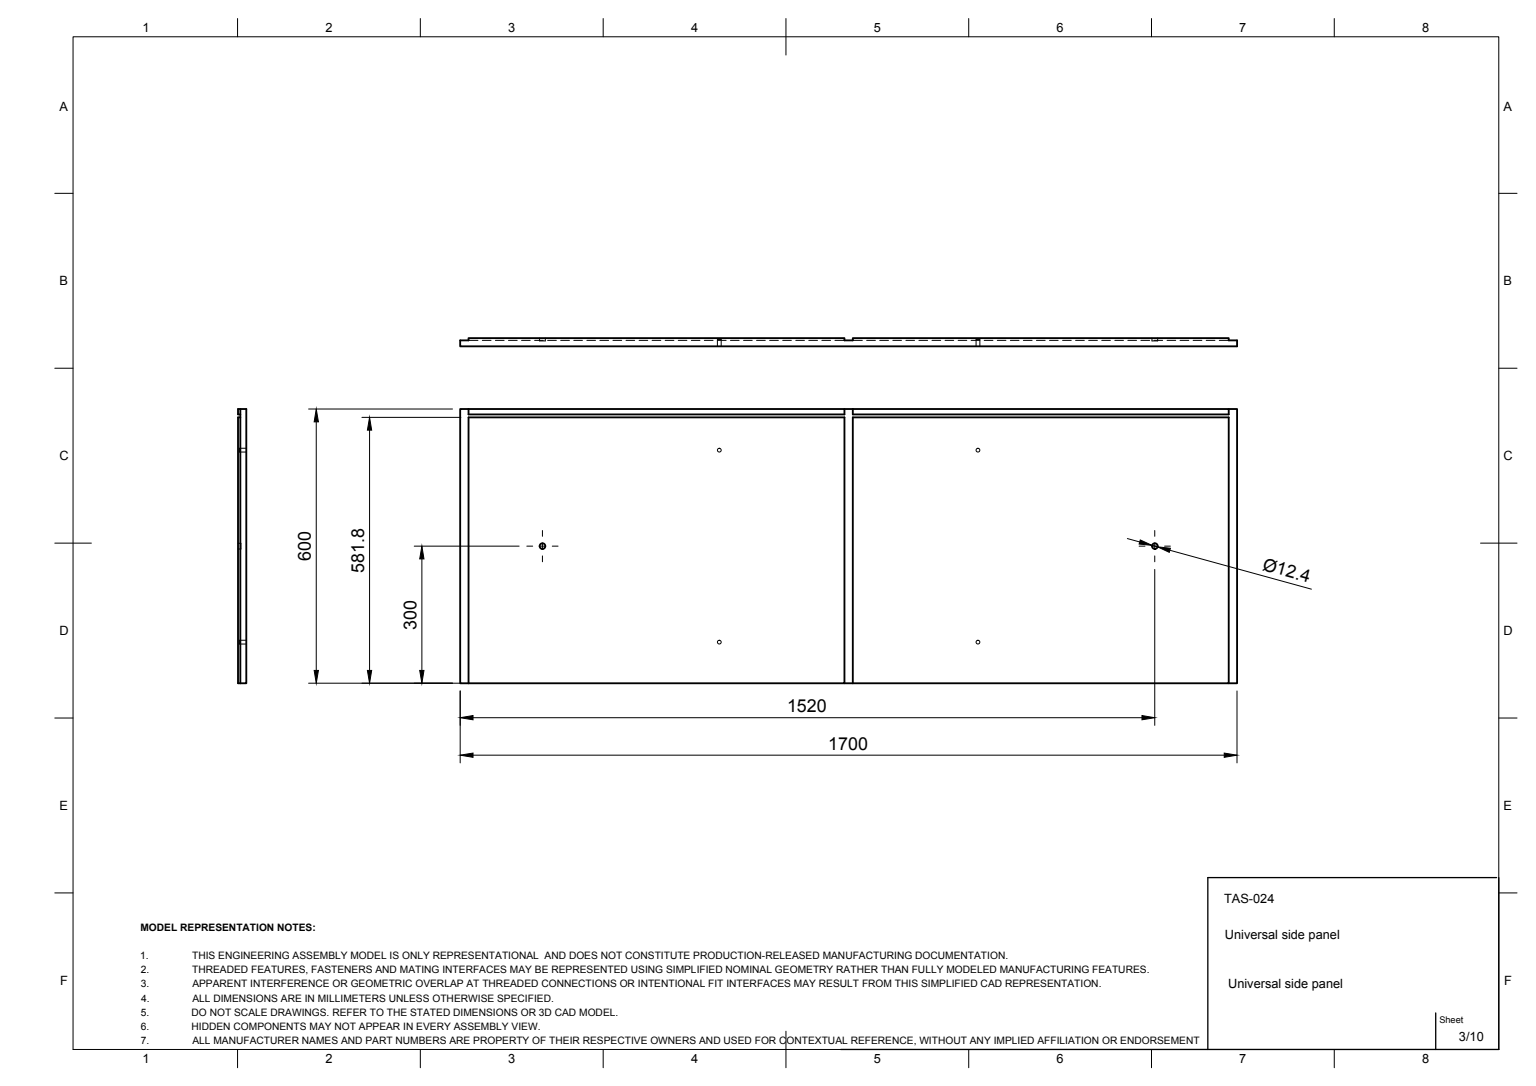
ISO-10303-21;
HEADER;
/* Generated by software containing ST-Developer
 * from STEP Tools, Inc. (www.steptools.com) 
 */

FILE_DESCRIPTION(
/* description */ (''),
/* implementation_level */ '2;1');

FILE_NAME(
/* name */ 'Universal side panel.step',
/* time_stamp */ '2026-11-15T17:53:25-08:00',
/* author */ (''),
/* organization */ (''),
/* preprocessor_version */ 'ST-DEVELOPER v20.2',
/* originating_system */ 'Autodesk Translation Framework v15.17.0.0',
/* authorisation */ '');

FILE_SCHEMA (('AUTOMOTIVE_DESIGN { 1 0 10303 214 3 1 1 }'));
ENDSEC;

DATA;
#10=MECHANICAL_DESIGN_GEOMETRIC_PRESENTATION_REPRESENTATION('',(#131),#2673);
#115=SHAPE_REPRESENTATION_RELATIONSHIP('SRR','None',#2723,#123);
#123=ADVANCED_BREP_SHAPE_REPRESENTATION('',(#139),#2665);
#131=STYLED_ITEM('',(#2772),#139);
#139=MANIFOLD_SOLID_BREP('Body1',#1517);
#147=FACE_BOUND('',#342,.T.);
#148=FACE_BOUND('',#349,.T.);
#149=FACE_BOUND('',#357,.T.);
#150=FACE_BOUND('',#358,.T.);
#151=FACE_BOUND('',#359,.T.);
#152=FACE_BOUND('',#360,.T.);
#160=PLANE('',#1619);
#161=PLANE('',#1623);
#162=PLANE('',#1627);
#163=PLANE('',#1631);
#164=PLANE('',#1635);
#165=PLANE('',#1639);
#166=PLANE('',#1640);
#167=PLANE('',#1641);
#168=PLANE('',#1642);
#169=PLANE('',#1643);
#170=PLANE('',#1644);
#171=PLANE('',#1645);
#172=PLANE('',#1646);
#173=PLANE('',#1647);
#174=PLANE('',#1648);
#175=PLANE('',#1649);
#176=PLANE('',#1650);
#177=PLANE('',#1651);
#178=PLANE('',#1652);
#179=PLANE('',#1653);
#180=PLANE('',#1654);
#181=PLANE('',#1655);
#182=PLANE('',#1656);
#183=PLANE('',#1657);
#184=PLANE('',#1658);
#185=PLANE('',#1659);
#186=PLANE('',#1660);
#187=PLANE('',#1661);
#233=FACE_OUTER_BOUND('',#322,.T.);
#234=FACE_OUTER_BOUND('',#323,.T.);
#235=FACE_OUTER_BOUND('',#324,.T.);
#236=FACE_OUTER_BOUND('',#325,.T.);
#237=FACE_OUTER_BOUND('',#326,.T.);
#238=FACE_OUTER_BOUND('',#327,.T.);
#239=FACE_OUTER_BOUND('',#328,.T.);
#240=FACE_OUTER_BOUND('',#329,.T.);
#241=FACE_OUTER_BOUND('',#330,.T.);
#242=FACE_OUTER_BOUND('',#331,.T.);
#243=FACE_OUTER_BOUND('',#332,.T.);
#244=FACE_OUTER_BOUND('',#333,.T.);
#245=FACE_OUTER_BOUND('',#334,.T.);
#246=FACE_OUTER_BOUND('',#335,.T.);
#247=FACE_OUTER_BOUND('',#336,.T.);
#248=FACE_OUTER_BOUND('',#337,.T.);
#249=FACE_OUTER_BOUND('',#338,.T.);
#250=FACE_OUTER_BOUND('',#339,.T.);
#251=FACE_OUTER_BOUND('',#340,.T.);
#252=FACE_OUTER_BOUND('',#341,.T.);
#253=FACE_OUTER_BOUND('',#343,.T.);
#254=FACE_OUTER_BOUND('',#344,.T.);
#255=FACE_OUTER_BOUND('',#345,.T.);
#256=FACE_OUTER_BOUND('',#346,.T.);
#257=FACE_OUTER_BOUND('',#347,.T.);
#258=FACE_OUTER_BOUND('',#348,.T.);
#259=FACE_OUTER_BOUND('',#350,.T.);
#260=FACE_OUTER_BOUND('',#351,.T.);
#261=FACE_OUTER_BOUND('',#352,.T.);
#262=FACE_OUTER_BOUND('',#353,.T.);
#263=FACE_OUTER_BOUND('',#354,.T.);
#264=FACE_OUTER_BOUND('',#355,.T.);
#265=FACE_OUTER_BOUND('',#356,.T.);
#266=FACE_OUTER_BOUND('',#361,.T.);
#322=EDGE_LOOP('',(#1052,#1053,#1054,#1055));
#323=EDGE_LOOP('',(#1056));
#324=EDGE_LOOP('',(#1057,#1058,#1059,#1060));
#325=EDGE_LOOP('',(#1061));
#326=EDGE_LOOP('',(#1062,#1063,#1064,#1065));
#327=EDGE_LOOP('',(#1066));
#328=EDGE_LOOP('',(#1067,#1068,#1069,#1070));
#329=EDGE_LOOP('',(#1071));
#330=EDGE_LOOP('',(#1072,#1073,#1074,#1075));
#331=EDGE_LOOP('',(#1076));
#332=EDGE_LOOP('',(#1077,#1078,#1079,#1080));
#333=EDGE_LOOP('',(#1081));
#334=EDGE_LOOP('',(#1082,#1083,#1084,#1085));
#335=EDGE_LOOP('',(#1086,#1087,#1088,#1089));
#336=EDGE_LOOP('',(#1090,#1091,#1092,#1093));
#337=EDGE_LOOP('',(#1094,#1095,#1096,#1097));
#338=EDGE_LOOP('',(#1098,#1099,#1100,#1101,#1102,#1103,#1104,#1105,#1106,
#1107,#1108,#1109,#1110,#1111,#1112,#1113,#1114,#1115,#1116,#1117));
#339=EDGE_LOOP('',(#1118,#1119,#1120,#1121));
#340=EDGE_LOOP('',(#1122,#1123,#1124,#1125));
#341=EDGE_LOOP('',(#1126,#1127,#1128,#1129));
#342=EDGE_LOOP('',(#1130));
#343=EDGE_LOOP('',(#1131,#1132,#1133,#1134));
#344=EDGE_LOOP('',(#1135,#1136,#1137,#1138));
#345=EDGE_LOOP('',(#1139,#1140,#1141,#1142));
#346=EDGE_LOOP('',(#1143,#1144,#1145,#1146));
#347=EDGE_LOOP('',(#1147,#1148,#1149,#1150));
#348=EDGE_LOOP('',(#1151,#1152,#1153,#1154));
#349=EDGE_LOOP('',(#1155));
#350=EDGE_LOOP('',(#1156,#1157,#1158,#1159));
#351=EDGE_LOOP('',(#1160,#1161,#1162,#1163));
#352=EDGE_LOOP('',(#1164,#1165,#1166,#1167));
#353=EDGE_LOOP('',(#1168,#1169,#1170,#1171,#1172,#1173,#1174,#1175,#1176,
#1177,#1178,#1179));
#354=EDGE_LOOP('',(#1180,#1181,#1182,#1183));
#355=EDGE_LOOP('',(#1184,#1185,#1186,#1187,#1188,#1189,#1190,#1191,#1192,
#1193,#1194,#1195));
#356=EDGE_LOOP('',(#1196,#1197,#1198,#1199));
#357=EDGE_LOOP('',(#1200));
#358=EDGE_LOOP('',(#1201));
#359=EDGE_LOOP('',(#1202));
#360=EDGE_LOOP('',(#1203));
#361=EDGE_LOOP('',(#1204,#1205,#1206,#1207));
#424=LINE('',#2236,#572);
#425=LINE('',#2243,#573);
#426=LINE('',#2250,#574);
#427=LINE('',#2257,#575);
#428=LINE('',#2264,#576);
#429=LINE('',#2271,#577);
#430=LINE('',#2277,#578);
#431=LINE('',#2279,#579);
#432=LINE('',#2281,#580);
#433=LINE('',#2282,#581);
#434=LINE('',#2286,#582);
#435=LINE('',#2288,#583);
#436=LINE('',#2290,#584);
#437=LINE('',#2291,#585);
#438=LINE('',#2295,#586);
#439=LINE('',#2297,#587);
#440=LINE('',#2299,#588);
#441=LINE('',#2300,#589);
#442=LINE('',#2304,#590);
#443=LINE('',#2306,#591);
#444=LINE('',#2308,#592);
#445=LINE('',#2309,#593);
#446=LINE('',#2312,#594);
#447=LINE('',#2314,#595);
#448=LINE('',#2316,#596);
#449=LINE('',#2318,#597);
#450=LINE('',#2319,#598);
#451=LINE('',#2321,#599);
#452=LINE('',#2323,#600);
#453=LINE('',#2324,#601);
#454=LINE('',#2326,#602);
#455=LINE('',#2328,#603);
#456=LINE('',#2330,#604);
#457=LINE('',#2332,#605);
#458=LINE('',#2333,#606);
#459=LINE('',#2335,#607);
#460=LINE('',#2337,#608);
#461=LINE('',#2338,#609);
#462=LINE('',#2341,#610);
#463=LINE('',#2342,#611);
#464=LINE('',#2345,#612);
#465=LINE('',#2346,#613);
#466=LINE('',#2349,#614);
#467=LINE('',#2350,#615);
#468=LINE('',#2353,#616);
#469=LINE('',#2354,#617);
#470=LINE('',#2356,#618);
#471=LINE('',#2358,#619);
#472=LINE('',#2361,#620);
#473=LINE('',#2362,#621);
#474=LINE('',#2365,#622);
#475=LINE('',#2366,#623);
#476=LINE('',#2369,#624);
#477=LINE('',#2370,#625);
#478=LINE('',#2373,#626);
#479=LINE('',#2374,#627);
#480=LINE('',#2376,#628);
#481=LINE('',#2378,#629);
#482=LINE('',#2381,#630);
#483=LINE('',#2383,#631);
#484=LINE('',#2384,#632);
#485=LINE('',#2387,#633);
#486=LINE('',#2388,#634);
#487=LINE('',#2391,#635);
#488=LINE('',#2392,#636);
#489=LINE('',#2394,#637);
#572=VECTOR('',#1778,0.409999999999997);
#573=VECTOR('',#1787,0.409999999999997);
#574=VECTOR('',#1796,0.409999999999997);
#575=VECTOR('',#1805,0.409999999999997);
#576=VECTOR('',#1814,0.620000000000001);
#577=VECTOR('',#1823,0.620000000000005);
#578=VECTOR('',#1830,1.);
#579=VECTOR('',#1831,1.);
#580=VECTOR('',#1832,1.);
#581=VECTOR('',#1833,1.);
#582=VECTOR('',#1836,1.);
#583=VECTOR('',#1837,1.);
#584=VECTOR('',#1838,1.);
#585=VECTOR('',#1839,1.);
#586=VECTOR('',#1842,1.);
#587=VECTOR('',#1843,1.);
#588=VECTOR('',#1844,1.);
#589=VECTOR('',#1845,1.);
#590=VECTOR('',#1848,1.);
#591=VECTOR('',#1849,1.);
#592=VECTOR('',#1850,1.);
#593=VECTOR('',#1851,1.);
#594=VECTOR('',#1854,1.);
#595=VECTOR('',#1855,1.);
#596=VECTOR('',#1856,1.);
#597=VECTOR('',#1857,1.);
#598=VECTOR('',#1858,1.);
#599=VECTOR('',#1859,1.);
#600=VECTOR('',#1860,1.);
#601=VECTOR('',#1861,1.);
#602=VECTOR('',#1862,1.);
#603=VECTOR('',#1863,1.);
#604=VECTOR('',#1864,1.);
#605=VECTOR('',#1865,1.);
#606=VECTOR('',#1866,1.);
#607=VECTOR('',#1867,1.);
#608=VECTOR('',#1868,1.);
#609=VECTOR('',#1869,1.);
#610=VECTOR('',#1872,1.);
#611=VECTOR('',#1873,1.);
#612=VECTOR('',#1876,1.);
#613=VECTOR('',#1877,1.);
#614=VECTOR('',#1880,1.);
#615=VECTOR('',#1881,1.);
#616=VECTOR('',#1884,1.);
#617=VECTOR('',#1885,1.);
#618=VECTOR('',#1888,1.);
#619=VECTOR('',#1891,1.);
#620=VECTOR('',#1894,1.);
#621=VECTOR('',#1895,1.);
#622=VECTOR('',#1898,1.);
#623=VECTOR('',#1899,1.);
#624=VECTOR('',#1902,1.);
#625=VECTOR('',#1903,1.);
#626=VECTOR('',#1906,1.);
#627=VECTOR('',#1907,1.);
#628=VECTOR('',#1910,1.);
#629=VECTOR('',#1913,1.);
#630=VECTOR('',#1916,1.);
#631=VECTOR('',#1917,1.);
#632=VECTOR('',#1918,1.);
#633=VECTOR('',#1921,1.);
#634=VECTOR('',#1922,1.);
#635=VECTOR('',#1925,1.);
#636=VECTOR('',#1926,1.);
#637=VECTOR('',#1929,1.);
#720=CIRCLE('',#1617,0.409999999999997);
#721=CIRCLE('',#1618,0.409999999999997);
#722=CIRCLE('',#1621,0.409999999999997);
#723=CIRCLE('',#1622,0.409999999999997);
#724=CIRCLE('',#1625,0.409999999999997);
#725=CIRCLE('',#1626,0.409999999999997);
#726=CIRCLE('',#1629,0.409999999999997);
#727=CIRCLE('',#1630,0.409999999999997);
#728=CIRCLE('',#1633,0.620000000000001);
#729=CIRCLE('',#1634,0.620000000000001);
#730=CIRCLE('',#1637,0.620000000000005);
#731=CIRCLE('',#1638,0.620000000000005);
#752=VERTEX_POINT('',#2233);
#753=VERTEX_POINT('',#2235);
#754=VERTEX_POINT('',#2240);
#755=VERTEX_POINT('',#2242);
#756=VERTEX_POINT('',#2247);
#757=VERTEX_POINT('',#2249);
#758=VERTEX_POINT('',#2254);
#759=VERTEX_POINT('',#2256);
#760=VERTEX_POINT('',#2261);
#761=VERTEX_POINT('',#2263);
#762=VERTEX_POINT('',#2268);
#763=VERTEX_POINT('',#2270);
#764=VERTEX_POINT('',#2275);
#765=VERTEX_POINT('',#2276);
#766=VERTEX_POINT('',#2278);
#767=VERTEX_POINT('',#2280);
#768=VERTEX_POINT('',#2284);
#769=VERTEX_POINT('',#2285);
#770=VERTEX_POINT('',#2287);
#771=VERTEX_POINT('',#2289);
#772=VERTEX_POINT('',#2293);
#773=VERTEX_POINT('',#2294);
#774=VERTEX_POINT('',#2296);
#775=VERTEX_POINT('',#2298);
#776=VERTEX_POINT('',#2302);
#777=VERTEX_POINT('',#2303);
#778=VERTEX_POINT('',#2305);
#779=VERTEX_POINT('',#2307);
#780=VERTEX_POINT('',#2311);
#781=VERTEX_POINT('',#2313);
#782=VERTEX_POINT('',#2315);
#783=VERTEX_POINT('',#2317);
#784=VERTEX_POINT('',#2320);
#785=VERTEX_POINT('',#2322);
#786=VERTEX_POINT('',#2325);
#787=VERTEX_POINT('',#2327);
#788=VERTEX_POINT('',#2329);
#789=VERTEX_POINT('',#2331);
#790=VERTEX_POINT('',#2334);
#791=VERTEX_POINT('',#2336);
#792=VERTEX_POINT('',#2340);
#793=VERTEX_POINT('',#2344);
#794=VERTEX_POINT('',#2348);
#795=VERTEX_POINT('',#2352);
#796=VERTEX_POINT('',#2360);
#797=VERTEX_POINT('',#2364);
#798=VERTEX_POINT('',#2368);
#799=VERTEX_POINT('',#2372);
#800=VERTEX_POINT('',#2380);
#801=VERTEX_POINT('',#2382);
#802=VERTEX_POINT('',#2386);
#803=VERTEX_POINT('',#2390);
#872=EDGE_CURVE('',#752,#752,#720,.T.);
#873=EDGE_CURVE('',#752,#753,#424,.T.);
#874=EDGE_CURVE('',#753,#753,#721,.T.);
#875=EDGE_CURVE('',#754,#754,#722,.T.);
#876=EDGE_CURVE('',#754,#755,#425,.T.);
#877=EDGE_CURVE('',#755,#755,#723,.T.);
#878=EDGE_CURVE('',#756,#756,#724,.T.);
#879=EDGE_CURVE('',#756,#757,#426,.T.);
#880=EDGE_CURVE('',#757,#757,#725,.T.);
#881=EDGE_CURVE('',#758,#758,#726,.T.);
#882=EDGE_CURVE('',#758,#759,#427,.T.);
#883=EDGE_CURVE('',#759,#759,#727,.T.);
#884=EDGE_CURVE('',#760,#760,#728,.T.);
#885=EDGE_CURVE('',#760,#761,#428,.T.);
#886=EDGE_CURVE('',#761,#761,#729,.T.);
#887=EDGE_CURVE('',#762,#762,#730,.T.);
#888=EDGE_CURVE('',#762,#763,#429,.T.);
#889=EDGE_CURVE('',#763,#763,#731,.T.);
#890=EDGE_CURVE('',#764,#765,#430,.T.);
#891=EDGE_CURVE('',#766,#764,#431,.T.);
#892=EDGE_CURVE('',#767,#766,#432,.T.);
#893=EDGE_CURVE('',#765,#767,#433,.T.);
#894=EDGE_CURVE('',#768,#769,#434,.T.);
#895=EDGE_CURVE('',#770,#768,#435,.T.);
#896=EDGE_CURVE('',#771,#770,#436,.T.);
#897=EDGE_CURVE('',#769,#771,#437,.T.);
#898=EDGE_CURVE('',#772,#773,#438,.T.);
#899=EDGE_CURVE('',#774,#772,#439,.T.);
#900=EDGE_CURVE('',#775,#774,#440,.T.);
#901=EDGE_CURVE('',#775,#773,#441,.T.);
#902=EDGE_CURVE('',#776,#777,#442,.T.);
#903=EDGE_CURVE('',#778,#776,#443,.T.);
#904=EDGE_CURVE('',#779,#778,#444,.T.);
#905=EDGE_CURVE('',#779,#777,#445,.T.);
#906=EDGE_CURVE('',#780,#768,#446,.T.);
#907=EDGE_CURVE('',#781,#780,#447,.T.);
#908=EDGE_CURVE('',#782,#781,#448,.T.);
#909=EDGE_CURVE('',#783,#782,#449,.T.);
#910=EDGE_CURVE('',#777,#783,#450,.T.);
#911=EDGE_CURVE('',#779,#784,#451,.T.);
#912=EDGE_CURVE('',#785,#784,#452,.T.);
#913=EDGE_CURVE('',#773,#785,#453,.T.);
#914=EDGE_CURVE('',#775,#786,#454,.T.);
#915=EDGE_CURVE('',#787,#786,#455,.T.);
#916=EDGE_CURVE('',#788,#787,#456,.T.);
#917=EDGE_CURVE('',#789,#788,#457,.T.);
#918=EDGE_CURVE('',#789,#766,#458,.T.);
#919=EDGE_CURVE('',#790,#764,#459,.T.);
#920=EDGE_CURVE('',#791,#790,#460,.T.);
#921=EDGE_CURVE('',#791,#770,#461,.T.);
#922=EDGE_CURVE('',#792,#783,#462,.T.);
#923=EDGE_CURVE('',#776,#792,#463,.T.);
#924=EDGE_CURVE('',#793,#769,#464,.T.);
#925=EDGE_CURVE('',#780,#793,#465,.T.);
#926=EDGE_CURVE('',#794,#792,#466,.T.);
#927=EDGE_CURVE('',#794,#778,#467,.T.);
#928=EDGE_CURVE('',#771,#795,#468,.T.);
#929=EDGE_CURVE('',#795,#793,#469,.T.);
#930=EDGE_CURVE('',#784,#794,#470,.T.);
#931=EDGE_CURVE('',#795,#791,#471,.T.);
#932=EDGE_CURVE('',#796,#785,#472,.T.);
#933=EDGE_CURVE('',#772,#796,#473,.T.);
#934=EDGE_CURVE('',#797,#765,#474,.T.);
#935=EDGE_CURVE('',#790,#797,#475,.T.);
#936=EDGE_CURVE('',#798,#796,#476,.T.);
#937=EDGE_CURVE('',#798,#774,#477,.T.);
#938=EDGE_CURVE('',#767,#799,#478,.T.);
#939=EDGE_CURVE('',#799,#797,#479,.T.);
#940=EDGE_CURVE('',#786,#798,#480,.T.);
#941=EDGE_CURVE('',#799,#789,#481,.T.);
#942=EDGE_CURVE('',#788,#800,#482,.T.);
#943=EDGE_CURVE('',#800,#801,#483,.T.);
#944=EDGE_CURVE('',#781,#801,#484,.T.);
#945=EDGE_CURVE('',#802,#787,#485,.T.);
#946=EDGE_CURVE('',#800,#802,#486,.T.);
#947=EDGE_CURVE('',#803,#782,#487,.T.);
#948=EDGE_CURVE('',#802,#803,#488,.T.);
#949=EDGE_CURVE('',#801,#803,#489,.T.);
#1052=ORIENTED_EDGE('',*,*,#872,.F.);
#1053=ORIENTED_EDGE('',*,*,#873,.T.);
#1054=ORIENTED_EDGE('',*,*,#874,.T.);
#1055=ORIENTED_EDGE('',*,*,#873,.F.);
#1056=ORIENTED_EDGE('',*,*,#874,.F.);
#1057=ORIENTED_EDGE('',*,*,#875,.F.);
#1058=ORIENTED_EDGE('',*,*,#876,.T.);
#1059=ORIENTED_EDGE('',*,*,#877,.T.);
#1060=ORIENTED_EDGE('',*,*,#876,.F.);
#1061=ORIENTED_EDGE('',*,*,#877,.F.);
#1062=ORIENTED_EDGE('',*,*,#878,.F.);
#1063=ORIENTED_EDGE('',*,*,#879,.T.);
#1064=ORIENTED_EDGE('',*,*,#880,.T.);
#1065=ORIENTED_EDGE('',*,*,#879,.F.);
#1066=ORIENTED_EDGE('',*,*,#880,.F.);
#1067=ORIENTED_EDGE('',*,*,#881,.F.);
#1068=ORIENTED_EDGE('',*,*,#882,.T.);
#1069=ORIENTED_EDGE('',*,*,#883,.T.);
#1070=ORIENTED_EDGE('',*,*,#882,.F.);
#1071=ORIENTED_EDGE('',*,*,#883,.F.);
#1072=ORIENTED_EDGE('',*,*,#884,.F.);
#1073=ORIENTED_EDGE('',*,*,#885,.T.);
#1074=ORIENTED_EDGE('',*,*,#886,.T.);
#1075=ORIENTED_EDGE('',*,*,#885,.F.);
#1076=ORIENTED_EDGE('',*,*,#886,.F.);
#1077=ORIENTED_EDGE('',*,*,#887,.F.);
#1078=ORIENTED_EDGE('',*,*,#888,.T.);
#1079=ORIENTED_EDGE('',*,*,#889,.T.);
#1080=ORIENTED_EDGE('',*,*,#888,.F.);
#1081=ORIENTED_EDGE('',*,*,#889,.F.);
#1082=ORIENTED_EDGE('',*,*,#890,.F.);
#1083=ORIENTED_EDGE('',*,*,#891,.F.);
#1084=ORIENTED_EDGE('',*,*,#892,.F.);
#1085=ORIENTED_EDGE('',*,*,#893,.F.);
#1086=ORIENTED_EDGE('',*,*,#894,.F.);
#1087=ORIENTED_EDGE('',*,*,#895,.F.);
#1088=ORIENTED_EDGE('',*,*,#896,.F.);
#1089=ORIENTED_EDGE('',*,*,#897,.F.);
#1090=ORIENTED_EDGE('',*,*,#898,.F.);
#1091=ORIENTED_EDGE('',*,*,#899,.F.);
#1092=ORIENTED_EDGE('',*,*,#900,.F.);
#1093=ORIENTED_EDGE('',*,*,#901,.T.);
#1094=ORIENTED_EDGE('',*,*,#902,.F.);
#1095=ORIENTED_EDGE('',*,*,#903,.F.);
#1096=ORIENTED_EDGE('',*,*,#904,.F.);
#1097=ORIENTED_EDGE('',*,*,#905,.T.);
#1098=ORIENTED_EDGE('',*,*,#906,.F.);
#1099=ORIENTED_EDGE('',*,*,#907,.F.);
#1100=ORIENTED_EDGE('',*,*,#908,.F.);
#1101=ORIENTED_EDGE('',*,*,#909,.F.);
#1102=ORIENTED_EDGE('',*,*,#910,.F.);
#1103=ORIENTED_EDGE('',*,*,#905,.F.);
#1104=ORIENTED_EDGE('',*,*,#911,.T.);
#1105=ORIENTED_EDGE('',*,*,#912,.F.);
#1106=ORIENTED_EDGE('',*,*,#913,.F.);
#1107=ORIENTED_EDGE('',*,*,#901,.F.);
#1108=ORIENTED_EDGE('',*,*,#914,.T.);
#1109=ORIENTED_EDGE('',*,*,#915,.F.);
#1110=ORIENTED_EDGE('',*,*,#916,.F.);
#1111=ORIENTED_EDGE('',*,*,#917,.F.);
#1112=ORIENTED_EDGE('',*,*,#918,.T.);
#1113=ORIENTED_EDGE('',*,*,#891,.T.);
#1114=ORIENTED_EDGE('',*,*,#919,.F.);
#1115=ORIENTED_EDGE('',*,*,#920,.F.);
#1116=ORIENTED_EDGE('',*,*,#921,.T.);
#1117=ORIENTED_EDGE('',*,*,#895,.T.);
#1118=ORIENTED_EDGE('',*,*,#902,.T.);
#1119=ORIENTED_EDGE('',*,*,#910,.T.);
#1120=ORIENTED_EDGE('',*,*,#922,.F.);
#1121=ORIENTED_EDGE('',*,*,#923,.F.);
#1122=ORIENTED_EDGE('',*,*,#894,.T.);
#1123=ORIENTED_EDGE('',*,*,#924,.F.);
#1124=ORIENTED_EDGE('',*,*,#925,.F.);
#1125=ORIENTED_EDGE('',*,*,#906,.T.);
#1126=ORIENTED_EDGE('',*,*,#903,.T.);
#1127=ORIENTED_EDGE('',*,*,#923,.T.);
#1128=ORIENTED_EDGE('',*,*,#926,.F.);
#1129=ORIENTED_EDGE('',*,*,#927,.T.);
#1130=ORIENTED_EDGE('',*,*,#887,.T.);
#1131=ORIENTED_EDGE('',*,*,#897,.T.);
#1132=ORIENTED_EDGE('',*,*,#928,.T.);
#1133=ORIENTED_EDGE('',*,*,#929,.T.);
#1134=ORIENTED_EDGE('',*,*,#924,.T.);
#1135=ORIENTED_EDGE('',*,*,#904,.T.);
#1136=ORIENTED_EDGE('',*,*,#927,.F.);
#1137=ORIENTED_EDGE('',*,*,#930,.F.);
#1138=ORIENTED_EDGE('',*,*,#911,.F.);
#1139=ORIENTED_EDGE('',*,*,#896,.T.);
#1140=ORIENTED_EDGE('',*,*,#921,.F.);
#1141=ORIENTED_EDGE('',*,*,#931,.F.);
#1142=ORIENTED_EDGE('',*,*,#928,.F.);
#1143=ORIENTED_EDGE('',*,*,#898,.T.);
#1144=ORIENTED_EDGE('',*,*,#913,.T.);
#1145=ORIENTED_EDGE('',*,*,#932,.F.);
#1146=ORIENTED_EDGE('',*,*,#933,.F.);
#1147=ORIENTED_EDGE('',*,*,#890,.T.);
#1148=ORIENTED_EDGE('',*,*,#934,.F.);
#1149=ORIENTED_EDGE('',*,*,#935,.F.);
#1150=ORIENTED_EDGE('',*,*,#919,.T.);
#1151=ORIENTED_EDGE('',*,*,#899,.T.);
#1152=ORIENTED_EDGE('',*,*,#933,.T.);
#1153=ORIENTED_EDGE('',*,*,#936,.F.);
#1154=ORIENTED_EDGE('',*,*,#937,.T.);
#1155=ORIENTED_EDGE('',*,*,#884,.T.);
#1156=ORIENTED_EDGE('',*,*,#893,.T.);
#1157=ORIENTED_EDGE('',*,*,#938,.T.);
#1158=ORIENTED_EDGE('',*,*,#939,.T.);
#1159=ORIENTED_EDGE('',*,*,#934,.T.);
#1160=ORIENTED_EDGE('',*,*,#900,.T.);
#1161=ORIENTED_EDGE('',*,*,#937,.F.);
#1162=ORIENTED_EDGE('',*,*,#940,.F.);
#1163=ORIENTED_EDGE('',*,*,#914,.F.);
#1164=ORIENTED_EDGE('',*,*,#892,.T.);
#1165=ORIENTED_EDGE('',*,*,#918,.F.);
#1166=ORIENTED_EDGE('',*,*,#941,.F.);
#1167=ORIENTED_EDGE('',*,*,#938,.F.);
#1168=ORIENTED_EDGE('',*,*,#931,.T.);
#1169=ORIENTED_EDGE('',*,*,#920,.T.);
#1170=ORIENTED_EDGE('',*,*,#935,.T.);
#1171=ORIENTED_EDGE('',*,*,#939,.F.);
#1172=ORIENTED_EDGE('',*,*,#941,.T.);
#1173=ORIENTED_EDGE('',*,*,#917,.T.);
#1174=ORIENTED_EDGE('',*,*,#942,.T.);
#1175=ORIENTED_EDGE('',*,*,#943,.T.);
#1176=ORIENTED_EDGE('',*,*,#944,.F.);
#1177=ORIENTED_EDGE('',*,*,#907,.T.);
#1178=ORIENTED_EDGE('',*,*,#925,.T.);
#1179=ORIENTED_EDGE('',*,*,#929,.F.);
#1180=ORIENTED_EDGE('',*,*,#916,.T.);
#1181=ORIENTED_EDGE('',*,*,#945,.F.);
#1182=ORIENTED_EDGE('',*,*,#946,.F.);
#1183=ORIENTED_EDGE('',*,*,#942,.F.);
#1184=ORIENTED_EDGE('',*,*,#930,.T.);
#1185=ORIENTED_EDGE('',*,*,#926,.T.);
#1186=ORIENTED_EDGE('',*,*,#922,.T.);
#1187=ORIENTED_EDGE('',*,*,#909,.T.);
#1188=ORIENTED_EDGE('',*,*,#947,.F.);
#1189=ORIENTED_EDGE('',*,*,#948,.F.);
#1190=ORIENTED_EDGE('',*,*,#945,.T.);
#1191=ORIENTED_EDGE('',*,*,#915,.T.);
#1192=ORIENTED_EDGE('',*,*,#940,.T.);
#1193=ORIENTED_EDGE('',*,*,#936,.T.);
#1194=ORIENTED_EDGE('',*,*,#932,.T.);
#1195=ORIENTED_EDGE('',*,*,#912,.T.);
#1196=ORIENTED_EDGE('',*,*,#946,.T.);
#1197=ORIENTED_EDGE('',*,*,#948,.T.);
#1198=ORIENTED_EDGE('',*,*,#949,.F.);
#1199=ORIENTED_EDGE('',*,*,#943,.F.);
#1200=ORIENTED_EDGE('',*,*,#872,.T.);
#1201=ORIENTED_EDGE('',*,*,#875,.T.);
#1202=ORIENTED_EDGE('',*,*,#878,.T.);
#1203=ORIENTED_EDGE('',*,*,#881,.T.);
#1204=ORIENTED_EDGE('',*,*,#908,.T.);
#1205=ORIENTED_EDGE('',*,*,#944,.T.);
#1206=ORIENTED_EDGE('',*,*,#949,.T.);
#1207=ORIENTED_EDGE('',*,*,#947,.T.);
#1412=CYLINDRICAL_SURFACE('',#1616,0.409999999999997);
#1413=CYLINDRICAL_SURFACE('',#1620,0.409999999999997);
#1414=CYLINDRICAL_SURFACE('',#1624,0.409999999999997);
#1415=CYLINDRICAL_SURFACE('',#1628,0.409999999999997);
#1416=CYLINDRICAL_SURFACE('',#1632,0.620000000000001);
#1417=CYLINDRICAL_SURFACE('',#1636,0.620000000000005);
#1428=ADVANCED_FACE('',(#233),#1412,.F.);
#1429=ADVANCED_FACE('',(#234),#160,.F.);
#1430=ADVANCED_FACE('',(#235),#1413,.F.);
#1431=ADVANCED_FACE('',(#236),#161,.F.);
#1432=ADVANCED_FACE('',(#237),#1414,.F.);
#1433=ADVANCED_FACE('',(#238),#162,.F.);
#1434=ADVANCED_FACE('',(#239),#1415,.F.);
#1435=ADVANCED_FACE('',(#240),#163,.F.);
#1436=ADVANCED_FACE('',(#241),#1416,.F.);
#1437=ADVANCED_FACE('',(#242),#164,.T.);
#1438=ADVANCED_FACE('',(#243),#1417,.F.);
#1439=ADVANCED_FACE('',(#244),#165,.T.);
#1440=ADVANCED_FACE('',(#245),#166,.F.);
#1441=ADVANCED_FACE('',(#246),#167,.F.);
#1442=ADVANCED_FACE('',(#247),#168,.F.);
#1443=ADVANCED_FACE('',(#248),#169,.F.);
#1444=ADVANCED_FACE('',(#249),#170,.F.);
#1445=ADVANCED_FACE('',(#250),#171,.T.);
#1446=ADVANCED_FACE('',(#251),#172,.T.);
#1447=ADVANCED_FACE('',(#252,#147),#173,.T.);
#1448=ADVANCED_FACE('',(#253),#174,.T.);
#1449=ADVANCED_FACE('',(#254),#175,.F.);
#1450=ADVANCED_FACE('',(#255),#176,.F.);
#1451=ADVANCED_FACE('',(#256),#177,.T.);
#1452=ADVANCED_FACE('',(#257),#178,.T.);
#1453=ADVANCED_FACE('',(#258,#148),#179,.T.);
#1454=ADVANCED_FACE('',(#259),#180,.T.);
#1455=ADVANCED_FACE('',(#260),#181,.F.);
#1456=ADVANCED_FACE('',(#261),#182,.F.);
#1457=ADVANCED_FACE('',(#262),#183,.T.);
#1458=ADVANCED_FACE('',(#263),#184,.F.);
#1459=ADVANCED_FACE('',(#264),#185,.T.);
#1460=ADVANCED_FACE('',(#265,#149,#150,#151,#152),#186,.T.);
#1461=ADVANCED_FACE('',(#266),#187,.T.);
#1517=CLOSED_SHELL('',(#1428,#1429,#1430,#1431,#1432,#1433,#1434,#1435,
#1436,#1437,#1438,#1439,#1440,#1441,#1442,#1443,#1444,#1445,#1446,#1447,
#1448,#1449,#1450,#1451,#1452,#1453,#1454,#1455,#1456,#1457,#1458,#1459,
#1460,#1461));
#1615=AXIS2_PLACEMENT_3D('',#2231,#1772,#1773);
#1616=AXIS2_PLACEMENT_3D('',#2232,#1774,#1775);
#1617=AXIS2_PLACEMENT_3D('',#2234,#1776,#1777);
#1618=AXIS2_PLACEMENT_3D('',#2237,#1779,#1780);
#1619=AXIS2_PLACEMENT_3D('',#2238,#1781,#1782);
#1620=AXIS2_PLACEMENT_3D('',#2239,#1783,#1784);
#1621=AXIS2_PLACEMENT_3D('',#2241,#1785,#1786);
#1622=AXIS2_PLACEMENT_3D('',#2244,#1788,#1789);
#1623=AXIS2_PLACEMENT_3D('',#2245,#1790,#1791);
#1624=AXIS2_PLACEMENT_3D('',#2246,#1792,#1793);
#1625=AXIS2_PLACEMENT_3D('',#2248,#1794,#1795);
#1626=AXIS2_PLACEMENT_3D('',#2251,#1797,#1798);
#1627=AXIS2_PLACEMENT_3D('',#2252,#1799,#1800);
#1628=AXIS2_PLACEMENT_3D('',#2253,#1801,#1802);
#1629=AXIS2_PLACEMENT_3D('',#2255,#1803,#1804);
#1630=AXIS2_PLACEMENT_3D('',#2258,#1806,#1807);
#1631=AXIS2_PLACEMENT_3D('',#2259,#1808,#1809);
#1632=AXIS2_PLACEMENT_3D('',#2260,#1810,#1811);
#1633=AXIS2_PLACEMENT_3D('',#2262,#1812,#1813);
#1634=AXIS2_PLACEMENT_3D('',#2265,#1815,#1816);
#1635=AXIS2_PLACEMENT_3D('',#2266,#1817,#1818);
#1636=AXIS2_PLACEMENT_3D('',#2267,#1819,#1820);
#1637=AXIS2_PLACEMENT_3D('',#2269,#1821,#1822);
#1638=AXIS2_PLACEMENT_3D('',#2272,#1824,#1825);
#1639=AXIS2_PLACEMENT_3D('',#2273,#1826,#1827);
#1640=AXIS2_PLACEMENT_3D('',#2274,#1828,#1829);
#1641=AXIS2_PLACEMENT_3D('',#2283,#1834,#1835);
#1642=AXIS2_PLACEMENT_3D('',#2292,#1840,#1841);
#1643=AXIS2_PLACEMENT_3D('',#2301,#1846,#1847);
#1644=AXIS2_PLACEMENT_3D('',#2310,#1852,#1853);
#1645=AXIS2_PLACEMENT_3D('',#2339,#1870,#1871);
#1646=AXIS2_PLACEMENT_3D('',#2343,#1874,#1875);
#1647=AXIS2_PLACEMENT_3D('',#2347,#1878,#1879);
#1648=AXIS2_PLACEMENT_3D('',#2351,#1882,#1883);
#1649=AXIS2_PLACEMENT_3D('',#2355,#1886,#1887);
#1650=AXIS2_PLACEMENT_3D('',#2357,#1889,#1890);
#1651=AXIS2_PLACEMENT_3D('',#2359,#1892,#1893);
#1652=AXIS2_PLACEMENT_3D('',#2363,#1896,#1897);
#1653=AXIS2_PLACEMENT_3D('',#2367,#1900,#1901);
#1654=AXIS2_PLACEMENT_3D('',#2371,#1904,#1905);
#1655=AXIS2_PLACEMENT_3D('',#2375,#1908,#1909);
#1656=AXIS2_PLACEMENT_3D('',#2377,#1911,#1912);
#1657=AXIS2_PLACEMENT_3D('',#2379,#1914,#1915);
#1658=AXIS2_PLACEMENT_3D('',#2385,#1919,#1920);
#1659=AXIS2_PLACEMENT_3D('',#2389,#1923,#1924);
#1660=AXIS2_PLACEMENT_3D('',#2393,#1927,#1928);
#1661=AXIS2_PLACEMENT_3D('',#2395,#1930,#1931);
#1772=DIRECTION('axis',(0.,0.,1.));
#1773=DIRECTION('refdir',(1.,0.,0.));
#1774=DIRECTION('center_axis',(1.,0.,0.));
#1775=DIRECTION('ref_axis',(0.,0.,-1.));
#1776=DIRECTION('center_axis',(1.,0.,0.));
#1777=DIRECTION('ref_axis',(0.,0.,-1.));
#1778=DIRECTION('',(1.,0.,0.));
#1779=DIRECTION('center_axis',(1.,0.,0.));
#1780=DIRECTION('ref_axis',(0.,0.,-1.));
#1781=DIRECTION('center_axis',(1.,0.,0.));
#1782=DIRECTION('ref_axis',(0.,0.,-1.));
#1783=DIRECTION('center_axis',(1.,0.,0.));
#1784=DIRECTION('ref_axis',(0.,0.,-1.));
#1785=DIRECTION('center_axis',(1.,0.,0.));
#1786=DIRECTION('ref_axis',(0.,0.,-1.));
#1787=DIRECTION('',(1.,0.,0.));
#1788=DIRECTION('center_axis',(1.,0.,0.));
#1789=DIRECTION('ref_axis',(0.,0.,-1.));
#1790=DIRECTION('center_axis',(1.,0.,0.));
#1791=DIRECTION('ref_axis',(0.,0.,-1.));
#1792=DIRECTION('center_axis',(1.,0.,0.));
#1793=DIRECTION('ref_axis',(0.,0.,-1.));
#1794=DIRECTION('center_axis',(1.,0.,0.));
#1795=DIRECTION('ref_axis',(0.,0.,-1.));
#1796=DIRECTION('',(1.,0.,0.));
#1797=DIRECTION('center_axis',(1.,0.,0.));
#1798=DIRECTION('ref_axis',(0.,0.,-1.));
#1799=DIRECTION('center_axis',(1.,0.,0.));
#1800=DIRECTION('ref_axis',(0.,0.,-1.));
#1801=DIRECTION('center_axis',(1.,0.,0.));
#1802=DIRECTION('ref_axis',(0.,0.,-1.));
#1803=DIRECTION('center_axis',(1.,0.,0.));
#1804=DIRECTION('ref_axis',(0.,0.,-1.));
#1805=DIRECTION('',(1.,0.,0.));
#1806=DIRECTION('center_axis',(1.,0.,0.));
#1807=DIRECTION('ref_axis',(0.,0.,-1.));
#1808=DIRECTION('center_axis',(1.,0.,0.));
#1809=DIRECTION('ref_axis',(0.,0.,-1.));
#1810=DIRECTION('center_axis',(-1.,0.,0.));
#1811=DIRECTION('ref_axis',(0.,0.,-1.));
#1812=DIRECTION('center_axis',(-1.,0.,0.));
#1813=DIRECTION('ref_axis',(0.,0.,-1.));
#1814=DIRECTION('',(-1.,0.,0.));
#1815=DIRECTION('center_axis',(-1.,0.,0.));
#1816=DIRECTION('ref_axis',(0.,0.,-1.));
#1817=DIRECTION('center_axis',(1.,0.,0.));
#1818=DIRECTION('ref_axis',(0.,0.,-1.));
#1819=DIRECTION('center_axis',(-1.,0.,0.));
#1820=DIRECTION('ref_axis',(0.,0.,-1.));
#1821=DIRECTION('center_axis',(-1.,0.,0.));
#1822=DIRECTION('ref_axis',(0.,0.,-1.));
#1823=DIRECTION('',(-1.,0.,0.));
#1824=DIRECTION('center_axis',(-1.,0.,0.));
#1825=DIRECTION('ref_axis',(0.,0.,-1.));
#1826=DIRECTION('center_axis',(1.,0.,0.));
#1827=DIRECTION('ref_axis',(0.,0.,-1.));
#1828=DIRECTION('center_axis',(0.,1.,0.));
#1829=DIRECTION('ref_axis',(-1.,0.,0.));
#1830=DIRECTION('',(1.,0.,0.));
#1831=DIRECTION('',(0.,0.,1.));
#1832=DIRECTION('',(-1.,0.,0.));
#1833=DIRECTION('',(0.,0.,-1.));
#1834=DIRECTION('center_axis',(0.,1.,0.));
#1835=DIRECTION('ref_axis',(-1.,0.,0.));
#1836=DIRECTION('',(1.,0.,0.));
#1837=DIRECTION('',(0.,0.,1.));
#1838=DIRECTION('',(-1.,0.,0.));
#1839=DIRECTION('',(0.,0.,-1.));
#1840=DIRECTION('center_axis',(0.,-1.,0.));
#1841=DIRECTION('ref_axis',(1.,0.,0.));
#1842=DIRECTION('',(-1.,0.,0.));
#1843=DIRECTION('',(0.,0.,1.));
#1844=DIRECTION('',(1.,0.,0.));
#1845=DIRECTION('',(0.,0.,1.));
#1846=DIRECTION('center_axis',(0.,-1.,0.));
#1847=DIRECTION('ref_axis',(1.,0.,0.));
#1848=DIRECTION('',(-1.,0.,0.));
#1849=DIRECTION('',(0.,0.,1.));
#1850=DIRECTION('',(1.,0.,0.));
#1851=DIRECTION('',(0.,0.,1.));
#1852=DIRECTION('center_axis',(-1.,0.,0.));
#1853=DIRECTION('ref_axis',(0.,-1.,0.));
#1854=DIRECTION('',(0.,-1.,0.));
#1855=DIRECTION('',(0.,0.,-1.));
#1856=DIRECTION('',(0.,1.,0.));
#1857=DIRECTION('',(0.,0.,1.));
#1858=DIRECTION('',(0.,-1.,0.));
#1859=DIRECTION('',(0.,-1.,0.));
#1860=DIRECTION('',(0.,0.,1.));
#1861=DIRECTION('',(0.,-1.,0.));
#1862=DIRECTION('',(0.,-1.,0.));
#1863=DIRECTION('',(0.,0.,1.));
#1864=DIRECTION('',(0.,-1.,0.));
#1865=DIRECTION('',(0.,0.,-1.));
#1866=DIRECTION('',(0.,-1.,0.));
#1867=DIRECTION('',(0.,-1.,0.));
#1868=DIRECTION('',(0.,0.,-1.));
#1869=DIRECTION('',(0.,-1.,0.));
#1870=DIRECTION('center_axis',(0.,0.,1.));
#1871=DIRECTION('ref_axis',(1.,0.,0.));
#1872=DIRECTION('',(-1.,0.,0.));
#1873=DIRECTION('',(0.,-1.,0.));
#1874=DIRECTION('center_axis',(0.,0.,1.));
#1875=DIRECTION('ref_axis',(1.,0.,0.));
#1876=DIRECTION('',(0.,-1.,0.));
#1877=DIRECTION('',(1.,0.,0.));
#1878=DIRECTION('center_axis',(1.,0.,0.));
#1879=DIRECTION('ref_axis',(0.,1.,0.));
#1880=DIRECTION('',(0.,0.,1.));
#1881=DIRECTION('',(0.,1.,0.));
#1882=DIRECTION('center_axis',(1.,0.,0.));
#1883=DIRECTION('ref_axis',(0.,1.,0.));
#1884=DIRECTION('',(0.,1.,0.));
#1885=DIRECTION('',(0.,0.,1.));
#1886=DIRECTION('center_axis',(0.,0.,1.));
#1887=DIRECTION('ref_axis',(1.,0.,0.));
#1888=DIRECTION('',(1.,0.,0.));
#1889=DIRECTION('center_axis',(0.,0.,1.));
#1890=DIRECTION('ref_axis',(1.,0.,0.));
#1891=DIRECTION('',(-1.,0.,0.));
#1892=DIRECTION('center_axis',(0.,0.,1.));
#1893=DIRECTION('ref_axis',(1.,0.,0.));
#1894=DIRECTION('',(-1.,0.,0.));
#1895=DIRECTION('',(0.,-1.,0.));
#1896=DIRECTION('center_axis',(0.,0.,1.));
#1897=DIRECTION('ref_axis',(1.,0.,0.));
#1898=DIRECTION('',(0.,-1.,0.));
#1899=DIRECTION('',(1.,0.,0.));
#1900=DIRECTION('center_axis',(1.,0.,0.));
#1901=DIRECTION('ref_axis',(0.,1.,0.));
#1902=DIRECTION('',(0.,0.,1.));
#1903=DIRECTION('',(0.,1.,0.));
#1904=DIRECTION('center_axis',(1.,0.,0.));
#1905=DIRECTION('ref_axis',(0.,1.,0.));
#1906=DIRECTION('',(0.,1.,0.));
#1907=DIRECTION('',(0.,0.,1.));
#1908=DIRECTION('center_axis',(0.,0.,1.));
#1909=DIRECTION('ref_axis',(1.,0.,0.));
#1910=DIRECTION('',(1.,0.,0.));
#1911=DIRECTION('center_axis',(0.,0.,1.));
#1912=DIRECTION('ref_axis',(1.,0.,0.));
#1913=DIRECTION('',(-1.,0.,0.));
#1914=DIRECTION('center_axis',(0.,1.,0.));
#1915=DIRECTION('ref_axis',(-1.,0.,0.));
#1916=DIRECTION('',(-1.,0.,0.));
#1917=DIRECTION('',(0.,0.,1.));
#1918=DIRECTION('',(-1.,0.,0.));
#1919=DIRECTION('center_axis',(0.,0.,1.));
#1920=DIRECTION('ref_axis',(1.,0.,0.));
#1921=DIRECTION('',(1.,0.,0.));
#1922=DIRECTION('',(0.,-1.,0.));
#1923=DIRECTION('center_axis',(0.,-1.,0.));
#1924=DIRECTION('ref_axis',(1.,0.,0.));
#1925=DIRECTION('',(1.,0.,0.));
#1926=DIRECTION('',(0.,0.,1.));
#1927=DIRECTION('center_axis',(-1.,0.,0.));
#1928=DIRECTION('ref_axis',(0.,-1.,0.));
#1929=DIRECTION('',(0.,-1.,0.));
#1930=DIRECTION('center_axis',(0.,0.,1.));
#1931=DIRECTION('ref_axis',(1.,0.,0.));
#2231=CARTESIAN_POINT('',(0.,0.,0.));
#2232=CARTESIAN_POINT('Origin',(0.,51.,56.7));
#2233=CARTESIAN_POINT('',(0.,51.,57.11));
#2234=CARTESIAN_POINT('Origin',(0.,51.,56.7));
#2235=CARTESIAN_POINT('',(1.5,51.,57.11));
#2236=CARTESIAN_POINT('',(0.,51.,57.11));
#2237=CARTESIAN_POINT('Origin',(1.5,51.,56.7));
#2238=CARTESIAN_POINT('Origin',(1.5,51.,56.7));
#2239=CARTESIAN_POINT('Origin',(0.,9.,113.3));
#2240=CARTESIAN_POINT('',(0.,9.,113.71));
#2241=CARTESIAN_POINT('Origin',(0.,9.,113.3));
#2242=CARTESIAN_POINT('',(1.5,9.,113.71));
#2243=CARTESIAN_POINT('',(0.,9.,113.71));
#2244=CARTESIAN_POINT('Origin',(1.5,9.,113.3));
#2245=CARTESIAN_POINT('Origin',(1.5,9.,113.3));
#2246=CARTESIAN_POINT('Origin',(0.,9.,56.7));
#2247=CARTESIAN_POINT('',(0.,9.,57.11));
#2248=CARTESIAN_POINT('Origin',(0.,9.,56.7));
#2249=CARTESIAN_POINT('',(1.5,9.,57.11));
#2250=CARTESIAN_POINT('',(0.,9.,57.11));
#2251=CARTESIAN_POINT('Origin',(1.5,9.,56.7));
#2252=CARTESIAN_POINT('Origin',(1.5,9.,56.7));
#2253=CARTESIAN_POINT('Origin',(0.,51.,113.3));
#2254=CARTESIAN_POINT('',(0.,51.,113.71));
#2255=CARTESIAN_POINT('Origin',(0.,51.,113.3));
#2256=CARTESIAN_POINT('',(1.5,51.,113.71));
#2257=CARTESIAN_POINT('',(0.,51.,113.71));
#2258=CARTESIAN_POINT('Origin',(1.5,51.,113.3));
#2259=CARTESIAN_POINT('Origin',(1.5,51.,113.3));
#2260=CARTESIAN_POINT('Origin',(1.8,30.,18.));
#2261=CARTESIAN_POINT('',(1.8,30.,18.62));
#2262=CARTESIAN_POINT('Origin',(1.8,30.,18.));
#2263=CARTESIAN_POINT('',(1.18,30.,18.62));
#2264=CARTESIAN_POINT('',(1.8,30.,18.62));
#2265=CARTESIAN_POINT('Origin',(1.18,30.,18.));
#2266=CARTESIAN_POINT('Origin',(1.18,30.,18.));
#2267=CARTESIAN_POINT('Origin',(1.8,30.,152.));
#2268=CARTESIAN_POINT('',(1.8,30.,152.62));
#2269=CARTESIAN_POINT('Origin',(1.8,30.,152.));
#2270=CARTESIAN_POINT('',(1.18,30.,152.62));
#2271=CARTESIAN_POINT('',(1.8,30.,152.62));
#2272=CARTESIAN_POINT('Origin',(1.18,30.,152.));
#2273=CARTESIAN_POINT('Origin',(1.18,30.,152.));
#2274=CARTESIAN_POINT('Origin',(1.81,58.82,0.));
#2275=CARTESIAN_POINT('',(1.3,58.82,84.08));
#2276=CARTESIAN_POINT('',(1.8,58.82,84.08));
#2277=CARTESIAN_POINT('',(1.6825,58.82,84.08));
#2278=CARTESIAN_POINT('',(1.3,58.82,1.82));
#2279=CARTESIAN_POINT('',(1.3,58.82,0.));
#2280=CARTESIAN_POINT('',(1.8,58.82,1.82));
#2281=CARTESIAN_POINT('',(1.6825,58.82,1.82));
#2282=CARTESIAN_POINT('',(1.8,58.82,0.));
#2283=CARTESIAN_POINT('Origin',(1.81,58.82,0.));
#2284=CARTESIAN_POINT('',(1.3,58.82,168.18));
#2285=CARTESIAN_POINT('',(1.8,58.82,168.18));
#2286=CARTESIAN_POINT('',(1.6825,58.82,168.18));
#2287=CARTESIAN_POINT('',(1.3,58.82,85.92));
#2288=CARTESIAN_POINT('',(1.3,58.82,0.));
#2289=CARTESIAN_POINT('',(1.8,58.82,85.92));
#2290=CARTESIAN_POINT('',(1.6825,58.82,85.92));
#2291=CARTESIAN_POINT('',(1.8,58.82,0.));
#2292=CARTESIAN_POINT('Origin',(1.3,58.18,0.));
#2293=CARTESIAN_POINT('',(1.8,58.18,84.08));
#2294=CARTESIAN_POINT('',(1.3,58.18,84.08));
#2295=CARTESIAN_POINT('',(1.4275,58.18,84.08));
#2296=CARTESIAN_POINT('',(1.8,58.18,1.82));
#2297=CARTESIAN_POINT('',(1.8,58.18,0.));
#2298=CARTESIAN_POINT('',(1.3,58.18,1.82));
#2299=CARTESIAN_POINT('',(1.4275,58.18,1.82));
#2300=CARTESIAN_POINT('',(1.3,58.18,0.));
#2301=CARTESIAN_POINT('Origin',(1.3,58.18,0.));
#2302=CARTESIAN_POINT('',(1.8,58.18,168.18));
#2303=CARTESIAN_POINT('',(1.3,58.18,168.18));
#2304=CARTESIAN_POINT('',(1.4275,58.18,168.18));
#2305=CARTESIAN_POINT('',(1.8,58.18,85.92));
#2306=CARTESIAN_POINT('',(1.8,58.18,0.));
#2307=CARTESIAN_POINT('',(1.3,58.18,85.92));
#2308=CARTESIAN_POINT('',(1.4275,58.18,85.92));
#2309=CARTESIAN_POINT('',(1.3,58.18,0.));
#2310=CARTESIAN_POINT('Origin',(1.3,60.,168.18));
#2311=CARTESIAN_POINT('',(1.3,60.,168.18));
#2312=CARTESIAN_POINT('',(1.3,60.,168.18));
#2313=CARTESIAN_POINT('',(1.3,60.,170.));
#2314=CARTESIAN_POINT('',(1.3,60.,84.09));
#2315=CARTESIAN_POINT('',(1.3,0.,170.));
#2316=CARTESIAN_POINT('',(1.3,45.,170.));
#2317=CARTESIAN_POINT('',(1.3,0.,168.18));
#2318=CARTESIAN_POINT('',(1.3,0.,84.09));
#2319=CARTESIAN_POINT('',(1.3,60.,168.18));
#2320=CARTESIAN_POINT('',(1.3,0.,85.92));
#2321=CARTESIAN_POINT('',(1.3,60.,85.92));
#2322=CARTESIAN_POINT('',(1.3,0.,84.08));
#2323=CARTESIAN_POINT('',(1.3,0.,42.04));
#2324=CARTESIAN_POINT('',(1.3,60.,84.08));
#2325=CARTESIAN_POINT('',(1.3,0.,1.82));
#2326=CARTESIAN_POINT('',(1.3,60.,1.82));
#2327=CARTESIAN_POINT('',(1.3,0.,0.));
#2328=CARTESIAN_POINT('',(1.3,0.,0.));
#2329=CARTESIAN_POINT('',(1.3,60.,0.));
#2330=CARTESIAN_POINT('',(1.3,45.,0.));
#2331=CARTESIAN_POINT('',(1.3,60.,1.82));
#2332=CARTESIAN_POINT('',(1.3,60.,0.));
#2333=CARTESIAN_POINT('',(1.3,60.,1.82));
#2334=CARTESIAN_POINT('',(1.3,60.,84.08));
#2335=CARTESIAN_POINT('',(1.3,60.,84.08));
#2336=CARTESIAN_POINT('',(1.3,60.,85.92));
#2337=CARTESIAN_POINT('',(1.3,60.,42.04));
#2338=CARTESIAN_POINT('',(1.3,60.,85.92));
#2339=CARTESIAN_POINT('Origin',(1.555,30.,168.18));
#2340=CARTESIAN_POINT('',(1.8,0.,168.18));
#2341=CARTESIAN_POINT('',(0.7775,0.,168.18));
#2342=CARTESIAN_POINT('',(1.8,15.,168.18));
#2343=CARTESIAN_POINT('Origin',(1.555,30.,168.18));
#2344=CARTESIAN_POINT('',(1.8,60.,168.18));
#2345=CARTESIAN_POINT('',(1.8,15.,168.18));
#2346=CARTESIAN_POINT('',(1.6775,60.,168.18));
#2347=CARTESIAN_POINT('Origin',(1.8,0.,0.));
#2348=CARTESIAN_POINT('',(1.8,0.,85.92));
#2349=CARTESIAN_POINT('',(1.8,0.,0.));
#2350=CARTESIAN_POINT('',(1.8,15.,85.92));
#2351=CARTESIAN_POINT('Origin',(1.8,0.,0.));
#2352=CARTESIAN_POINT('',(1.8,60.,85.92));
#2353=CARTESIAN_POINT('',(1.8,15.,85.92));
#2354=CARTESIAN_POINT('',(1.8,60.,0.));
#2355=CARTESIAN_POINT('Origin',(1.555,30.,85.92));
#2356=CARTESIAN_POINT('',(0.7775,0.,85.92));
#2357=CARTESIAN_POINT('Origin',(1.555,30.,85.92));
#2358=CARTESIAN_POINT('',(1.6775,60.,85.92));
#2359=CARTESIAN_POINT('Origin',(1.555,30.,84.08));
#2360=CARTESIAN_POINT('',(1.8,0.,84.08));
#2361=CARTESIAN_POINT('',(0.7775,0.,84.08));
#2362=CARTESIAN_POINT('',(1.8,15.,84.08));
#2363=CARTESIAN_POINT('Origin',(1.555,30.,84.08));
#2364=CARTESIAN_POINT('',(1.8,60.,84.08));
#2365=CARTESIAN_POINT('',(1.8,15.,84.08));
#2366=CARTESIAN_POINT('',(1.6775,60.,84.08));
#2367=CARTESIAN_POINT('Origin',(1.8,0.,0.));
#2368=CARTESIAN_POINT('',(1.8,0.,1.82));
#2369=CARTESIAN_POINT('',(1.8,0.,0.));
#2370=CARTESIAN_POINT('',(1.8,15.,1.82));
#2371=CARTESIAN_POINT('Origin',(1.8,0.,0.));
#2372=CARTESIAN_POINT('',(1.8,60.,1.82));
#2373=CARTESIAN_POINT('',(1.8,15.,1.82));
#2374=CARTESIAN_POINT('',(1.8,60.,0.));
#2375=CARTESIAN_POINT('Origin',(1.555,30.,1.82));
#2376=CARTESIAN_POINT('',(0.7775,0.,1.82));
#2377=CARTESIAN_POINT('Origin',(1.555,30.,1.82));
#2378=CARTESIAN_POINT('',(1.6775,60.,1.82));
#2379=CARTESIAN_POINT('Origin',(1.8,60.,0.));
#2380=CARTESIAN_POINT('',(0.,60.,0.));
#2381=CARTESIAN_POINT('',(1.8,60.,0.));
#2382=CARTESIAN_POINT('',(0.,60.,170.));
#2383=CARTESIAN_POINT('',(0.,60.,0.));
#2384=CARTESIAN_POINT('',(1.8,60.,170.));
#2385=CARTESIAN_POINT('Origin',(0.9,30.,0.));
#2386=CARTESIAN_POINT('',(0.,0.,0.));
#2387=CARTESIAN_POINT('',(0.,0.,0.));
#2388=CARTESIAN_POINT('',(0.,60.,0.));
#2389=CARTESIAN_POINT('Origin',(0.,0.,0.));
#2390=CARTESIAN_POINT('',(0.,0.,170.));
#2391=CARTESIAN_POINT('',(0.,0.,170.));
#2392=CARTESIAN_POINT('',(0.,0.,0.));
#2393=CARTESIAN_POINT('Origin',(0.,60.,0.));
#2394=CARTESIAN_POINT('',(0.,60.,170.));
#2395=CARTESIAN_POINT('Origin',(0.9,30.,170.));
#2655=UNCERTAINTY_MEASURE_WITH_UNIT(LENGTH_MEASURE(0.001),#2674,
'DISTANCE_ACCURACY_VALUE',
'Maximum model space distance between geometric entities at asserted c
onnectivities');
#2663=UNCERTAINTY_MEASURE_WITH_UNIT(LENGTH_MEASURE(0.001),#2674,
'DISTANCE_ACCURACY_VALUE',
'Maximum model space distance between geometric entities at asserted c
onnectivities');
#2665=(
GEOMETRIC_REPRESENTATION_CONTEXT(3)
GLOBAL_UNCERTAINTY_ASSIGNED_CONTEXT((#2655))
GLOBAL_UNIT_ASSIGNED_CONTEXT((#2674,#2676,#2677))
REPRESENTATION_CONTEXT('','3D')
);
#2673=(
GEOMETRIC_REPRESENTATION_CONTEXT(3)
GLOBAL_UNCERTAINTY_ASSIGNED_CONTEXT((#2663))
GLOBAL_UNIT_ASSIGNED_CONTEXT((#2674,#2676,#2677))
REPRESENTATION_CONTEXT('','3D')
);
#2674=(
LENGTH_UNIT()
NAMED_UNIT(*)
SI_UNIT(.CENTI.,.METRE.)
);
#2676=(
NAMED_UNIT(*)
PLANE_ANGLE_UNIT()
SI_UNIT($,.RADIAN.)
);
#2677=(
NAMED_UNIT(*)
SI_UNIT($,.STERADIAN.)
SOLID_ANGLE_UNIT()
);
#2679=SHAPE_DEFINITION_REPRESENTATION(#2688,#2723);
#2688=PRODUCT_DEFINITION_SHAPE('',$,#2733);
#2723=SHAPE_REPRESENTATION('',(#1615),#2665);
#2731=PRODUCT_DEFINITION_CONTEXT('part definition',#2760,'design');
#2733=PRODUCT_DEFINITION('Universal side panel','Universal side panel',
#2742,#2731);
#2742=PRODUCT_DEFINITION_FORMATION('',$,#2763);
#2760=APPLICATION_CONTEXT(
'Core Data for Automotive Mechanical Design Process');
#2761=PRODUCT_CONTEXT('part definition',#2760,'mechanical');
#2763=PRODUCT('Universal side panel','Universal side panel',$,(#2761));
#2772=PRESENTATION_STYLE_ASSIGNMENT((#2781));
#2781=SURFACE_STYLE_USAGE(.BOTH.,#2790);
#2790=SURFACE_SIDE_STYLE('',(#2799));
#2799=SURFACE_STYLE_FILL_AREA(#2808);
#2808=FILL_AREA_STYLE('Universal side panel finish',(#2817));
#2817=FILL_AREA_STYLE_COLOUR('Universal side panel finish',#2826);
#2826=COLOUR_RGB('Universal side panel finish',0.0941176470588235,0.231372549019608,
0.431372549019608);
ENDSEC;
END-ISO-10303-21;
